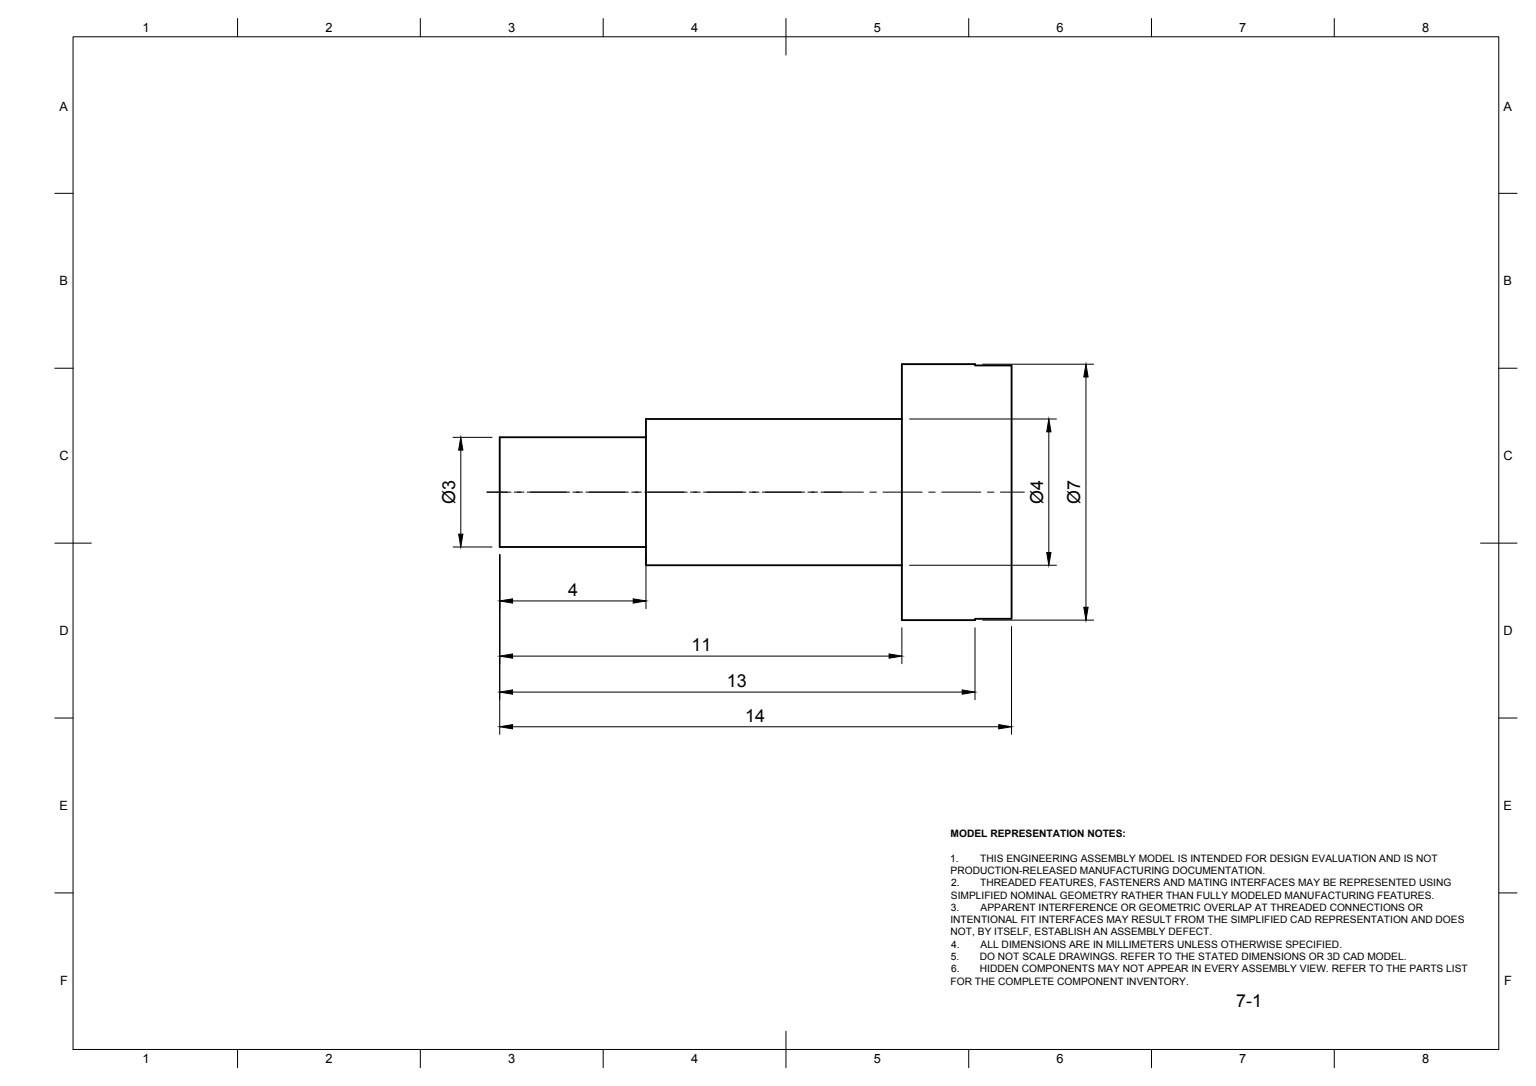
ISO-10303-21;
HEADER;
/* Generated by software containing ST-Developer
 * from STEP Tools, Inc. (www.steptools.com) 
 */

FILE_DESCRIPTION(
/* description */ (''),
/* implementation_level */ '2;1');

FILE_NAME(
/* name */ '7-1.step',
/* time_stamp */ '2026-10-06T01:16:10-07:00',
/* author */ (''),
/* organization */ (''),
/* preprocessor_version */ 'ST-DEVELOPER v20.2',
/* originating_system */ 'Autodesk Translation Framework v15.15.0.0',
/* authorisation */ '');

FILE_SCHEMA (('AUTOMOTIVE_DESIGN { 1 0 10303 214 3 1 1 }'));
ENDSEC;

DATA;
#10=MECHANICAL_DESIGN_GEOMETRIC_PRESENTATION_REPRESENTATION('',(#309,#310),#17113);
#228=OPEN_SHELL('',(#5877,#5878));
#246=SHELL_BASED_SURFACE_MODEL('Body2',(#228));
#270=SHAPE_REPRESENTATION_RELATIONSHIP('SRR','None',#17194,#286);
#286=ADVANCED_BREP_SHAPE_REPRESENTATION('',(#336),#17101);
#309=STYLED_ITEM('',(#17298),#336);
#310=STYLED_ITEM('',(#17298),#246);
#336=MANIFOLD_SOLID_BREP('Body1',#6022);
#441=CYLINDRICAL_SURFACE('',#6655,1.5);
#442=CYLINDRICAL_SURFACE('',#6659,2.);
#443=CYLINDRICAL_SURFACE('',#6663,3.5);
#444=CYLINDRICAL_SURFACE('',#6674,1.25);
#583=FACE_BOUND('',#1660,.T.);
#584=FACE_BOUND('',#1663,.T.);
#585=FACE_BOUND('',#1672,.T.);
#856=CIRCLE('',#6654,1.5);
#857=CIRCLE('',#6656,1.5);
#858=CIRCLE('',#6658,2.);
#859=CIRCLE('',#6660,2.);
#860=CIRCLE('',#6662,3.5);
#861=CIRCLE('',#6664,3.5);
#862=CIRCLE('',#6665,3.5);
#863=CIRCLE('',#6666,3.5);
#864=CIRCLE('',#6667,3.5);
#865=CIRCLE('',#6668,3.5);
#866=CIRCLE('',#6675,1.25);
#867=CIRCLE('',#6676,1.25);
#868=CIRCLE('',#6678,1.5);
#1218=FACE_OUTER_BOUND('',#1657,.T.);
#1219=FACE_OUTER_BOUND('',#1658,.T.);
#1220=FACE_OUTER_BOUND('',#1659,.T.);
#1221=FACE_OUTER_BOUND('',#1661,.T.);
#1222=FACE_OUTER_BOUND('',#1662,.T.);
#1223=FACE_OUTER_BOUND('',#1664,.T.);
#1224=FACE_OUTER_BOUND('',#1665,.T.);
#1225=FACE_OUTER_BOUND('',#1666,.T.);
#1226=FACE_OUTER_BOUND('',#1667,.T.);
#1227=FACE_OUTER_BOUND('',#1668,.T.);
#1228=FACE_OUTER_BOUND('',#1669,.T.);
#1229=FACE_OUTER_BOUND('',#1670,.T.);
#1230=FACE_OUTER_BOUND('',#1671,.T.);
#1657=EDGE_LOOP('',(#4892));
#1658=EDGE_LOOP('',(#4893,#4894,#4895,#4896));
#1659=EDGE_LOOP('',(#4897));
#1660=EDGE_LOOP('',(#4898));
#1661=EDGE_LOOP('',(#4899,#4900,#4901,#4902));
#1662=EDGE_LOOP('',(#4903));
#1663=EDGE_LOOP('',(#4904));
#1664=EDGE_LOOP('',(#4905,#4906,#4907,#4908,#4909,#4910,#4911,#4912,#4913,
#4914,#4915,#4916));
#1665=EDGE_LOOP('',(#4917,#4918,#4919,#4920));
#1666=EDGE_LOOP('',(#4921,#4922,#4923,#4924));
#1667=EDGE_LOOP('',(#4925,#4926,#4927,#4928));
#1668=EDGE_LOOP('',(#4929,#4930));
#1669=EDGE_LOOP('',(#4931,#4932,#4933));
#1670=EDGE_LOOP('',(#4934,#4935,#4936,#4937));
#1671=EDGE_LOOP('',(#4938));
#1672=EDGE_LOOP('',(#4939));
#2088=LINE('',#10954,#2449);
#2089=LINE('',#10961,#2450);
#2090=LINE('',#10968,#2451);
#2091=LINE('',#10972,#2452);
#2092=LINE('',#10976,#2453);
#2093=LINE('',#10980,#2454);
#2094=LINE('',#10984,#2455);
#2095=LINE('',#10987,#2456);
#2096=LINE('',#10988,#2457);
#2097=LINE('',#10990,#2458);
#2098=LINE('',#10992,#2459);
#2099=LINE('',#10999,#2460);
#2449=VECTOR('',#8100,1.5);
#2450=VECTOR('',#8109,2.);
#2451=VECTOR('',#8118,3.5);
#2452=VECTOR('',#8121,1.);
#2453=VECTOR('',#8124,1.);
#2454=VECTOR('',#8127,1.);
#2455=VECTOR('',#8130,1.);
#2456=VECTOR('',#8135,6.928203230276);
#2457=VECTOR('',#8136,6.928203230276);
#2458=VECTOR('',#8139,6.928203230276);
#2459=VECTOR('',#8142,6.928203230276);
#2460=VECTOR('',#8151,1.25);
#2892=VERTEX_POINT('',#10950);
#2893=VERTEX_POINT('',#10953);
#2894=VERTEX_POINT('',#10957);
#2895=VERTEX_POINT('',#10960);
#2896=VERTEX_POINT('',#10964);
#2897=VERTEX_POINT('',#10967);
#2898=VERTEX_POINT('',#10969);
#2899=VERTEX_POINT('',#10971);
#2900=VERTEX_POINT('',#10973);
#2901=VERTEX_POINT('',#10975);
#2902=VERTEX_POINT('',#10977);
#2903=VERTEX_POINT('',#10979);
#2904=VERTEX_POINT('',#10981);
#2905=VERTEX_POINT('',#10983);
#2906=VERTEX_POINT('',#10996);
#2907=VERTEX_POINT('',#10998);
#2908=VERTEX_POINT('',#11002);
#3599=EDGE_CURVE('',#2892,#2892,#856,.T.);
#3600=EDGE_CURVE('',#2892,#2893,#2088,.T.);
#3601=EDGE_CURVE('',#2893,#2893,#857,.T.);
#3602=EDGE_CURVE('',#2894,#2894,#858,.T.);
#3603=EDGE_CURVE('',#2894,#2895,#2089,.T.);
#3604=EDGE_CURVE('',#2895,#2895,#859,.T.);
#3605=EDGE_CURVE('',#2896,#2896,#860,.T.);
#3606=EDGE_CURVE('',#2896,#2897,#2090,.T.);
#3607=EDGE_CURVE('',#2897,#2898,#861,.T.);
#3608=EDGE_CURVE('',#2898,#2899,#2091,.T.);
#3609=EDGE_CURVE('',#2899,#2900,#862,.T.);
#3610=EDGE_CURVE('',#2901,#2900,#2092,.T.);
#3611=EDGE_CURVE('',#2902,#2901,#863,.T.);
#3612=EDGE_CURVE('',#2902,#2903,#2093,.T.);
#3613=EDGE_CURVE('',#2903,#2904,#864,.T.);
#3614=EDGE_CURVE('',#2905,#2904,#2094,.T.);
#3615=EDGE_CURVE('',#2905,#2897,#865,.T.);
#3616=EDGE_CURVE('',#2903,#2900,#2095,.T.);
#3617=EDGE_CURVE('',#2901,#2902,#2096,.T.);
#3618=EDGE_CURVE('',#2904,#2899,#2097,.T.);
#3619=EDGE_CURVE('',#2898,#2905,#2098,.T.);
#3620=EDGE_CURVE('',#2906,#2906,#866,.T.);
#3621=EDGE_CURVE('',#2906,#2907,#2099,.T.);
#3622=EDGE_CURVE('',#2907,#2907,#867,.T.);
#3623=EDGE_CURVE('',#2908,#2908,#868,.T.);
#4892=ORIENTED_EDGE('',*,*,#3599,.F.);
#4893=ORIENTED_EDGE('',*,*,#3599,.T.);
#4894=ORIENTED_EDGE('',*,*,#3600,.T.);
#4895=ORIENTED_EDGE('',*,*,#3601,.T.);
#4896=ORIENTED_EDGE('',*,*,#3600,.F.);
#4897=ORIENTED_EDGE('',*,*,#3602,.F.);
#4898=ORIENTED_EDGE('',*,*,#3601,.F.);
#4899=ORIENTED_EDGE('',*,*,#3602,.T.);
#4900=ORIENTED_EDGE('',*,*,#3603,.T.);
#4901=ORIENTED_EDGE('',*,*,#3604,.T.);
#4902=ORIENTED_EDGE('',*,*,#3603,.F.);
#4903=ORIENTED_EDGE('',*,*,#3605,.F.);
#4904=ORIENTED_EDGE('',*,*,#3604,.F.);
#4905=ORIENTED_EDGE('',*,*,#3605,.T.);
#4906=ORIENTED_EDGE('',*,*,#3606,.T.);
#4907=ORIENTED_EDGE('',*,*,#3607,.T.);
#4908=ORIENTED_EDGE('',*,*,#3608,.T.);
#4909=ORIENTED_EDGE('',*,*,#3609,.T.);
#4910=ORIENTED_EDGE('',*,*,#3610,.F.);
#4911=ORIENTED_EDGE('',*,*,#3611,.F.);
#4912=ORIENTED_EDGE('',*,*,#3612,.T.);
#4913=ORIENTED_EDGE('',*,*,#3613,.T.);
#4914=ORIENTED_EDGE('',*,*,#3614,.F.);
#4915=ORIENTED_EDGE('',*,*,#3615,.T.);
#4916=ORIENTED_EDGE('',*,*,#3606,.F.);
#4917=ORIENTED_EDGE('',*,*,#3610,.T.);
#4918=ORIENTED_EDGE('',*,*,#3616,.F.);
#4919=ORIENTED_EDGE('',*,*,#3612,.F.);
#4920=ORIENTED_EDGE('',*,*,#3617,.F.);
#4921=ORIENTED_EDGE('',*,*,#3609,.F.);
#4922=ORIENTED_EDGE('',*,*,#3618,.F.);
#4923=ORIENTED_EDGE('',*,*,#3613,.F.);
#4924=ORIENTED_EDGE('',*,*,#3616,.T.);
#4925=ORIENTED_EDGE('',*,*,#3608,.F.);
#4926=ORIENTED_EDGE('',*,*,#3619,.T.);
#4927=ORIENTED_EDGE('',*,*,#3614,.T.);
#4928=ORIENTED_EDGE('',*,*,#3618,.T.);
#4929=ORIENTED_EDGE('',*,*,#3617,.T.);
#4930=ORIENTED_EDGE('',*,*,#3611,.T.);
#4931=ORIENTED_EDGE('',*,*,#3619,.F.);
#4932=ORIENTED_EDGE('',*,*,#3607,.F.);
#4933=ORIENTED_EDGE('',*,*,#3615,.F.);
#4934=ORIENTED_EDGE('',*,*,#3620,.F.);
#4935=ORIENTED_EDGE('',*,*,#3621,.T.);
#4936=ORIENTED_EDGE('',*,*,#3622,.T.);
#4937=ORIENTED_EDGE('',*,*,#3621,.F.);
#4938=ORIENTED_EDGE('',*,*,#3623,.F.);
#4939=ORIENTED_EDGE('',*,*,#3622,.F.);
#5583=PLANE('',#6653);
#5584=PLANE('',#6657);
#5585=PLANE('',#6661);
#5586=PLANE('',#6669);
#5587=PLANE('',#6670);
#5588=PLANE('',#6671);
#5589=PLANE('',#6672);
#5590=PLANE('',#6673);
#5591=PLANE('',#6677);
#5866=ADVANCED_FACE('',(#1218),#5583,.T.);
#5867=ADVANCED_FACE('',(#1219),#441,.T.);
#5868=ADVANCED_FACE('',(#1220,#583),#5584,.T.);
#5869=ADVANCED_FACE('',(#1221),#442,.T.);
#5870=ADVANCED_FACE('',(#1222,#584),#5585,.T.);
#5871=ADVANCED_FACE('',(#1223),#443,.T.);
#5872=ADVANCED_FACE('',(#1224),#5586,.F.);
#5873=ADVANCED_FACE('',(#1225),#5587,.F.);
#5874=ADVANCED_FACE('',(#1226),#5588,.F.);
#5875=ADVANCED_FACE('',(#1227),#5589,.F.);
#5876=ADVANCED_FACE('',(#1228),#5590,.F.);
#5877=ADVANCED_FACE('',(#1229),#444,.T.);
#5878=ADVANCED_FACE('',(#1230,#585),#5591,.T.);
#6022=CLOSED_SHELL('',(#5866,#5867,#5868,#5869,#5870,#5871,#5872,#5873,
#5874,#5875,#5876));
#6652=AXIS2_PLACEMENT_3D('',#10948,#8092,#8093);
#6653=AXIS2_PLACEMENT_3D('',#10949,#8094,#8095);
#6654=AXIS2_PLACEMENT_3D('',#10951,#8096,#8097);
#6655=AXIS2_PLACEMENT_3D('',#10952,#8098,#8099);
#6656=AXIS2_PLACEMENT_3D('',#10955,#8101,#8102);
#6657=AXIS2_PLACEMENT_3D('',#10956,#8103,#8104);
#6658=AXIS2_PLACEMENT_3D('',#10958,#8105,#8106);
#6659=AXIS2_PLACEMENT_3D('',#10959,#8107,#8108);
#6660=AXIS2_PLACEMENT_3D('',#10962,#8110,#8111);
#6661=AXIS2_PLACEMENT_3D('',#10963,#8112,#8113);
#6662=AXIS2_PLACEMENT_3D('',#10965,#8114,#8115);
#6663=AXIS2_PLACEMENT_3D('',#10966,#8116,#8117);
#6664=AXIS2_PLACEMENT_3D('',#10970,#8119,#8120);
#6665=AXIS2_PLACEMENT_3D('',#10974,#8122,#8123);
#6666=AXIS2_PLACEMENT_3D('',#10978,#8125,#8126);
#6667=AXIS2_PLACEMENT_3D('',#10982,#8128,#8129);
#6668=AXIS2_PLACEMENT_3D('',#10985,#8131,#8132);
#6669=AXIS2_PLACEMENT_3D('',#10986,#8133,#8134);
#6670=AXIS2_PLACEMENT_3D('',#10989,#8137,#8138);
#6671=AXIS2_PLACEMENT_3D('',#10991,#8140,#8141);
#6672=AXIS2_PLACEMENT_3D('',#10993,#8143,#8144);
#6673=AXIS2_PLACEMENT_3D('',#10994,#8145,#8146);
#6674=AXIS2_PLACEMENT_3D('',#10995,#8147,#8148);
#6675=AXIS2_PLACEMENT_3D('',#10997,#8149,#8150);
#6676=AXIS2_PLACEMENT_3D('',#11000,#8152,#8153);
#6677=AXIS2_PLACEMENT_3D('',#11001,#8154,#8155);
#6678=AXIS2_PLACEMENT_3D('',#11003,#8156,#8157);
#8092=DIRECTION('axis',(0.,0.,1.));
#8093=DIRECTION('refdir',(1.,0.,0.));
#8094=DIRECTION('center_axis',(0.,-1.,0.));
#8095=DIRECTION('ref_axis',(0.,0.,1.));
#8096=DIRECTION('center_axis',(0.,1.,0.));
#8097=DIRECTION('ref_axis',(0.,0.,-1.));
#8098=DIRECTION('center_axis',(0.,-1.,0.));
#8099=DIRECTION('ref_axis',(0.,0.,1.));
#8100=DIRECTION('',(0.,1.,0.));
#8101=DIRECTION('center_axis',(0.,-1.,0.));
#8102=DIRECTION('ref_axis',(0.,0.,-1.));
#8103=DIRECTION('center_axis',(0.,-1.,0.));
#8104=DIRECTION('ref_axis',(0.,0.,1.));
#8105=DIRECTION('center_axis',(0.,1.,0.));
#8106=DIRECTION('ref_axis',(0.,0.,-1.));
#8107=DIRECTION('center_axis',(0.,-1.,0.));
#8108=DIRECTION('ref_axis',(0.,0.,1.));
#8109=DIRECTION('',(0.,1.,0.));
#8110=DIRECTION('center_axis',(0.,-1.,0.));
#8111=DIRECTION('ref_axis',(0.,0.,-1.));
#8112=DIRECTION('center_axis',(0.,-1.,0.));
#8113=DIRECTION('ref_axis',(0.,0.,1.));
#8114=DIRECTION('center_axis',(0.,1.,0.));
#8115=DIRECTION('ref_axis',(0.,0.,-1.));
#8116=DIRECTION('center_axis',(0.,-1.,0.));
#8117=DIRECTION('ref_axis',(0.,0.,1.));
#8118=DIRECTION('',(0.,1.,0.));
#8119=DIRECTION('center_axis',(0.,-1.,0.));
#8120=DIRECTION('ref_axis',(0.,0.,-1.));
#8121=DIRECTION('',(0.,-1.,0.));
#8122=DIRECTION('center_axis',(0.,-1.,0.));
#8123=DIRECTION('ref_axis',(0.989743318610793,0.,-0.142857142857099));
#8124=DIRECTION('',(0.,-1.,0.));
#8125=DIRECTION('center_axis',(0.,1.,0.));
#8126=DIRECTION('ref_axis',(-0.989743318610793,0.,0.142857142857099));
#8127=DIRECTION('',(0.,-1.,0.));
#8128=DIRECTION('center_axis',(0.,-1.,0.));
#8129=DIRECTION('ref_axis',(-0.989743318610793,0.,0.142857142857099));
#8130=DIRECTION('',(0.,-1.,0.));
#8131=DIRECTION('center_axis',(0.,-1.,0.));
#8132=DIRECTION('ref_axis',(0.,0.,-1.));
#8133=DIRECTION('center_axis',(0.,0.,1.));
#8134=DIRECTION('ref_axis',(0.,-1.,0.));
#8135=DIRECTION('',(1.,0.,0.));
#8136=DIRECTION('',(-1.,0.,0.));
#8137=DIRECTION('center_axis',(0.,-1.,0.));
#8138=DIRECTION('ref_axis',(0.,0.,-1.));
#8139=DIRECTION('',(1.,0.,0.));
#8140=DIRECTION('center_axis',(0.,0.,-1.));
#8141=DIRECTION('ref_axis',(0.,1.,0.));
#8142=DIRECTION('',(-1.,0.,0.));
#8143=DIRECTION('center_axis',(0.,-1.,0.));
#8144=DIRECTION('ref_axis',(0.,0.,1.));
#8145=DIRECTION('center_axis',(0.,-1.,0.));
#8146=DIRECTION('ref_axis',(0.,0.,1.));
#8147=DIRECTION('center_axis',(0.,-1.,0.));
#8148=DIRECTION('ref_axis',(1.,0.,0.));
#8149=DIRECTION('center_axis',(0.,-1.,0.));
#8150=DIRECTION('ref_axis',(-1.,0.,0.));
#8151=DIRECTION('',(0.,1.,0.));
#8152=DIRECTION('center_axis',(0.,-1.,0.));
#8153=DIRECTION('ref_axis',(-1.,0.,0.));
#8154=DIRECTION('center_axis',(0.,-1.,0.));
#8155=DIRECTION('ref_axis',(1.,0.,0.));
#8156=DIRECTION('center_axis',(0.,1.,0.));
#8157=DIRECTION('ref_axis',(-1.,0.,0.));
#10948=CARTESIAN_POINT('',(0.,0.,0.));
#10949=CARTESIAN_POINT('Origin',(0.,-14.,0.));
#10950=CARTESIAN_POINT('',(1.83697019872103E-16,-14.,-1.5));
#10951=CARTESIAN_POINT('Origin',(0.,-14.,0.));
#10952=CARTESIAN_POINT('Origin',(0.,0.7,0.));
#10953=CARTESIAN_POINT('',(1.83697019872103E-16,-10.,-1.5));
#10954=CARTESIAN_POINT('',(1.83697019872103E-16,0.7,-1.5));
#10955=CARTESIAN_POINT('Origin',(0.,-10.,0.));
#10956=CARTESIAN_POINT('Origin',(0.,-10.,0.));
#10957=CARTESIAN_POINT('',(2.44929359829471E-16,-10.,-2.));
#10958=CARTESIAN_POINT('Origin',(0.,-10.,0.));
#10959=CARTESIAN_POINT('Origin',(0.,0.7,0.));
#10960=CARTESIAN_POINT('',(2.44929359829471E-16,-3.,-2.));
#10961=CARTESIAN_POINT('',(2.44929359829471E-16,0.7,-2.));
#10962=CARTESIAN_POINT('Origin',(0.,-3.,0.));
#10963=CARTESIAN_POINT('Origin',(0.,-3.,0.));
#10964=CARTESIAN_POINT('',(4.28626379701574E-16,-3.,-3.5));
#10965=CARTESIAN_POINT('Origin',(0.,-3.,0.));
#10966=CARTESIAN_POINT('Origin',(0.,0.7,0.));
#10967=CARTESIAN_POINT('',(4.28626379701574E-16,0.,-3.5));
#10968=CARTESIAN_POINT('',(4.28626379701574E-16,0.7,-3.5));
#10969=CARTESIAN_POINT('',(3.464101615138,0.,-0.5));
#10970=CARTESIAN_POINT('Origin',(0.,0.,0.));
#10971=CARTESIAN_POINT('',(3.464101615138,-1.,-0.5));
#10972=CARTESIAN_POINT('',(3.464101615138,0.,-0.5));
#10973=CARTESIAN_POINT('',(3.464101615138,-1.,0.5));
#10974=CARTESIAN_POINT('Origin',(0.,-1.,0.));
#10975=CARTESIAN_POINT('',(3.464101615138,0.,0.5));
#10976=CARTESIAN_POINT('',(3.464101615138,0.,0.5));
#10977=CARTESIAN_POINT('',(-3.464101615138,0.,0.5));
#10978=CARTESIAN_POINT('Origin',(0.,0.,0.));
#10979=CARTESIAN_POINT('',(-3.464101615138,-1.,0.5));
#10980=CARTESIAN_POINT('',(-3.464101615138,0.,0.5));
#10981=CARTESIAN_POINT('',(-3.464101615138,-1.,-0.5));
#10982=CARTESIAN_POINT('Origin',(0.,-1.,0.));
#10983=CARTESIAN_POINT('',(-3.464101615138,0.,-0.5));
#10984=CARTESIAN_POINT('',(-3.464101615138,0.,-0.5));
#10985=CARTESIAN_POINT('Origin',(0.,0.,0.));
#10986=CARTESIAN_POINT('Origin',(-5.15,0.,0.5));
#10987=CARTESIAN_POINT('',(-3.464101615138,-1.,0.5));
#10988=CARTESIAN_POINT('',(3.464101615138,0.,0.5));
#10989=CARTESIAN_POINT('Origin',(-5.15,-1.,0.5));
#10990=CARTESIAN_POINT('',(-3.464101615138,-1.,-0.5));
#10991=CARTESIAN_POINT('Origin',(-5.15,-1.,-0.5));
#10992=CARTESIAN_POINT('',(3.464101615138,0.,-0.5));
#10993=CARTESIAN_POINT('Origin',(0.,0.,0.));
#10994=CARTESIAN_POINT('Origin',(0.,0.,0.));
#10995=CARTESIAN_POINT('Origin',(0.,-14.,0.));
#10996=CARTESIAN_POINT('',(-1.25,-14.,-1.53080849893419E-16));
#10997=CARTESIAN_POINT('Origin',(0.,-14.,0.));
#10998=CARTESIAN_POINT('',(-1.25,-10.,-1.53080849893419E-16));
#10999=CARTESIAN_POINT('',(-1.25,-14.,-1.53080849893419E-16));
#11000=CARTESIAN_POINT('Origin',(0.,-10.,0.));
#11001=CARTESIAN_POINT('Origin',(0.,-10.,0.));
#11002=CARTESIAN_POINT('',(1.5,-10.,0.));
#11003=CARTESIAN_POINT('Origin',(0.,-10.,0.));
#17078=UNCERTAINTY_MEASURE_WITH_UNIT(LENGTH_MEASURE(0.01),#17114,
'DISTANCE_ACCURACY_VALUE',
'Maximum model space distance between geometric entities at asserted c
onnectivities');
#17090=UNCERTAINTY_MEASURE_WITH_UNIT(LENGTH_MEASURE(0.01),#17114,
'DISTANCE_ACCURACY_VALUE',
'Maximum model space distance between geometric entities at asserted c
onnectivities');
#17101=(
GEOMETRIC_REPRESENTATION_CONTEXT(3)
GLOBAL_UNCERTAINTY_ASSIGNED_CONTEXT((#17078))
GLOBAL_UNIT_ASSIGNED_CONTEXT((#17114,#17116,#17117))
REPRESENTATION_CONTEXT('','3D')
);
#17113=(
GEOMETRIC_REPRESENTATION_CONTEXT(3)
GLOBAL_UNCERTAINTY_ASSIGNED_CONTEXT((#17090))
GLOBAL_UNIT_ASSIGNED_CONTEXT((#17114,#17116,#17117))
REPRESENTATION_CONTEXT('','3D')
);
#17114=(
LENGTH_UNIT()
NAMED_UNIT(*)
SI_UNIT(.MILLI.,.METRE.)
);
#17116=(
NAMED_UNIT(*)
PLANE_ANGLE_UNIT()
SI_UNIT($,.RADIAN.)
);
#17117=(
NAMED_UNIT(*)
SI_UNIT($,.STERADIAN.)
SOLID_ANGLE_UNIT()
);
#17128=SHAPE_DEFINITION_REPRESENTATION(#17154,#17194);
#17154=PRODUCT_DEFINITION_SHAPE('',$,#17217);
#17194=SHAPE_REPRESENTATION('',(#6652,#246),#17101);
#17206=PRODUCT_DEFINITION_CONTEXT('part definition',#17274,'design');
#17217=PRODUCT_DEFINITION('7-1','7-1',#17239,#17206);
#17239=PRODUCT_DEFINITION_FORMATION('',$,#17286);
#17274=APPLICATION_CONTEXT(
'Core Data for Automotive Mechanical Design Process');
#17275=PRODUCT_CONTEXT('part definition',#17274,'mechanical');
#17286=PRODUCT('7-1','7-1','NOT SPECIFIED',(#17275));
#17298=PRESENTATION_STYLE_ASSIGNMENT((#17299));
#17299=SURFACE_STYLE_USAGE(.BOTH.,#17300);
#17300=SURFACE_SIDE_STYLE('',(#17301));
#17301=SURFACE_STYLE_FILL_AREA(#17302);
#17302=FILL_AREA_STYLE('Steel - Satin',(#17303));
#17303=FILL_AREA_STYLE_COLOUR('Steel - Satin',#17304);
#17304=COLOUR_RGB('Steel - Satin', 0.09019608, 0.27058824, 0.51372549);
ENDSEC;
END-ISO-10303-21;
